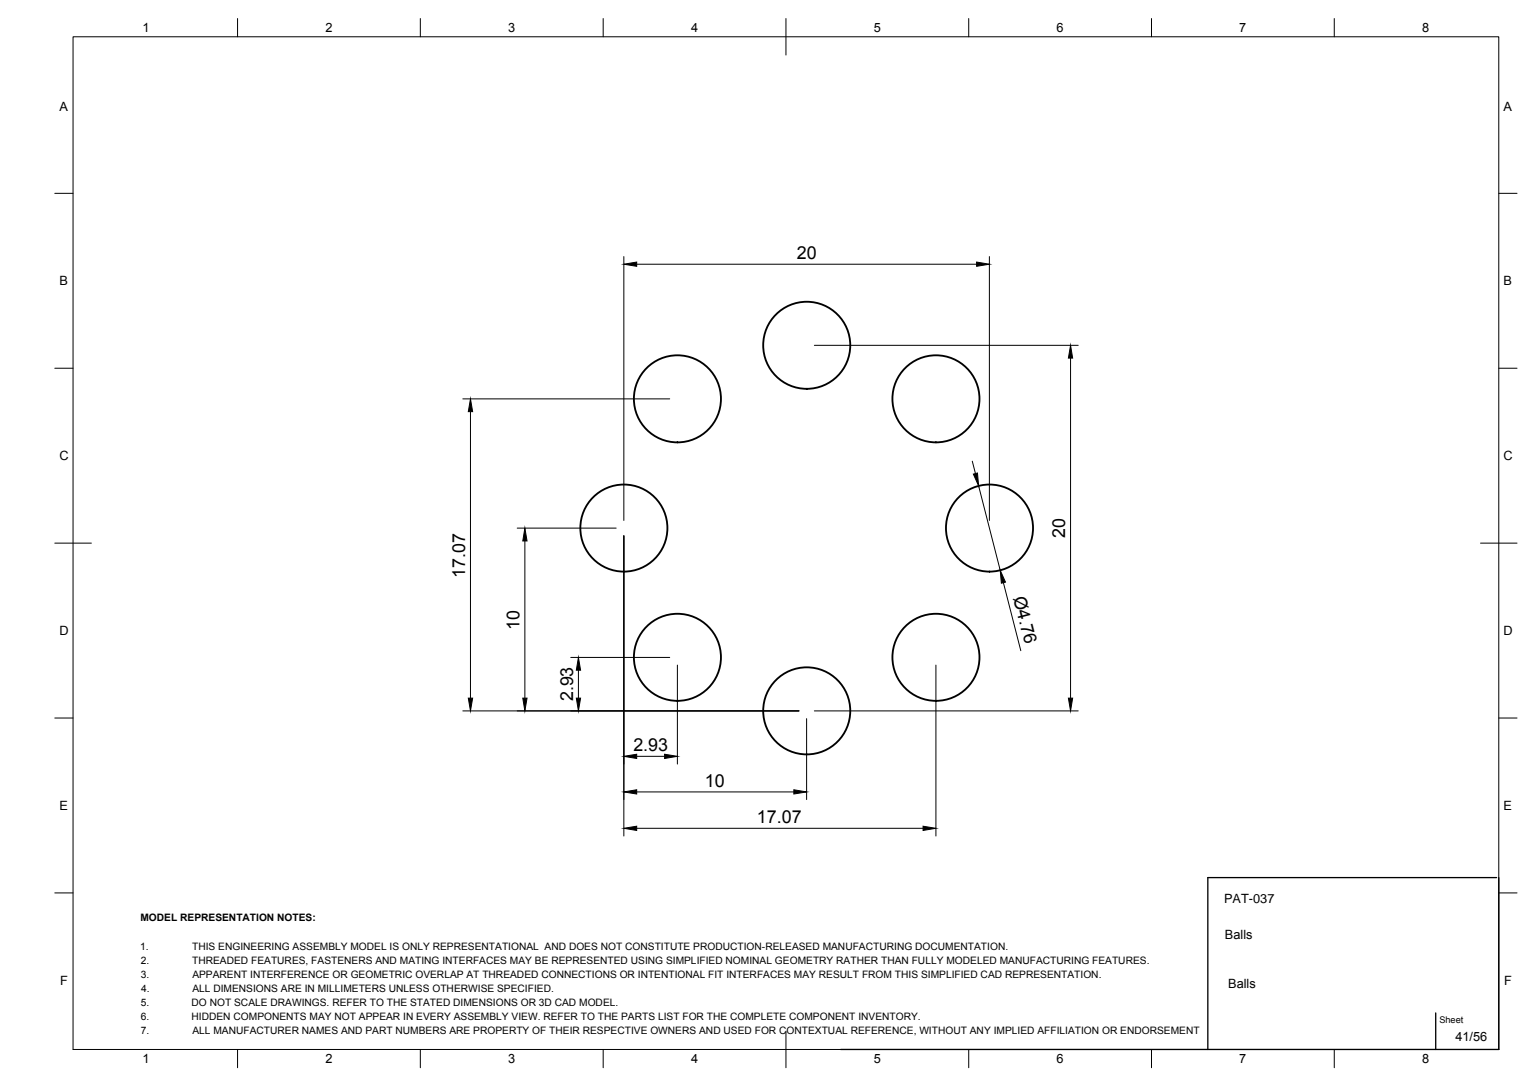
ISO-10303-21;
HEADER;
/* Generated by software containing ST-Developer
 * from STEP Tools, Inc. (www.steptools.com) 
 */

FILE_DESCRIPTION(
/* description */ ('Flywheel Crank-Slider'),
/* implementation_level */ '2;1');

FILE_NAME(
/* name */ 'Balls.step',
/* time_stamp */ '2026-10-28T03:23:13-07:00',
/* author */ (''),
/* organization */ (''),
/* preprocessor_version */ 'ST-DEVELOPER v20.2',
/* originating_system */ 'Autodesk Translation Framework v15.17.0.0',
/* authorisation */ '');

FILE_SCHEMA (('AUTOMOTIVE_DESIGN { 1 0 10303 214 3 1 1 }'));
ENDSEC;

DATA;
#10=MECHANICAL_DESIGN_GEOMETRIC_PRESENTATION_REPRESENTATION('',(#708,#709,#710,#711,#712,#713,#714,#715),#17322);
#513=SPHERICAL_SURFACE('',#10435,0.23815);
#514=SPHERICAL_SURFACE('',#10437,0.23815);
#515=SPHERICAL_SURFACE('',#10439,0.23815);
#516=SPHERICAL_SURFACE('',#10441,0.23815);
#517=SPHERICAL_SURFACE('',#10443,0.23815);
#518=SPHERICAL_SURFACE('',#10445,0.23815);
#519=SPHERICAL_SURFACE('',#10447,0.23815);
#520=SPHERICAL_SURFACE('',#10449,0.23815);
#603=SHAPE_REPRESENTATION_RELATIONSHIP('SRR','None',#17603,#655);
#655=ADVANCED_BREP_SHAPE_REPRESENTATION('',(#765,#766,#767,#768,#769,#770,
#771,#772),#17307);
#708=STYLED_ITEM('',(#17931),#765);
#709=STYLED_ITEM('',(#17931),#766);
#710=STYLED_ITEM('',(#17931),#767);
#711=STYLED_ITEM('',(#17931),#768);
#712=STYLED_ITEM('',(#17931),#769);
#713=STYLED_ITEM('',(#17931),#770);
#714=STYLED_ITEM('',(#17931),#771);
#715=STYLED_ITEM('',(#17931),#772);
#765=MANIFOLD_SOLID_BREP('Body1',#9090);
#766=MANIFOLD_SOLID_BREP('Body2',#9091);
#767=MANIFOLD_SOLID_BREP('Body3',#9092);
#768=MANIFOLD_SOLID_BREP('Body4',#9093);
#769=MANIFOLD_SOLID_BREP('Body5',#9094);
#770=MANIFOLD_SOLID_BREP('Body6',#9095);
#771=MANIFOLD_SOLID_BREP('Body7',#9096);
#772=MANIFOLD_SOLID_BREP('Body8',#9097);
#1718=FACE_OUTER_BOUND('',#2415,.T.);
#1719=FACE_OUTER_BOUND('',#2416,.T.);
#1720=FACE_OUTER_BOUND('',#2417,.T.);
#1721=FACE_OUTER_BOUND('',#2418,.T.);
#1722=FACE_OUTER_BOUND('',#2419,.T.);
#1723=FACE_OUTER_BOUND('',#2420,.T.);
#1724=FACE_OUTER_BOUND('',#2421,.T.);
#1725=FACE_OUTER_BOUND('',#2422,.T.);
#2415=EDGE_LOOP('',(#7762,#7763));
#2416=EDGE_LOOP('',(#7764,#7765));
#2417=EDGE_LOOP('',(#7766,#7767));
#2418=EDGE_LOOP('',(#7768,#7769));
#2419=EDGE_LOOP('',(#7770,#7771));
#2420=EDGE_LOOP('',(#7772,#7773));
#2421=EDGE_LOOP('',(#7774,#7775));
#2422=EDGE_LOOP('',(#7776,#7777));
#4142=CIRCLE('',#10436,0.23815);
#4143=CIRCLE('',#10438,0.23815);
#4144=CIRCLE('',#10440,0.23815);
#4145=CIRCLE('',#10442,0.23815);
#4146=CIRCLE('',#10444,0.23815);
#4147=CIRCLE('',#10446,0.23815);
#4148=CIRCLE('',#10448,0.23815);
#4149=CIRCLE('',#10450,0.23815);
#4819=VERTEX_POINT('',#16121);
#4820=VERTEX_POINT('',#16122);
#4821=VERTEX_POINT('',#16125);
#4822=VERTEX_POINT('',#16126);
#4823=VERTEX_POINT('',#16129);
#4824=VERTEX_POINT('',#16130);
#4825=VERTEX_POINT('',#16133);
#4826=VERTEX_POINT('',#16134);
#4827=VERTEX_POINT('',#16137);
#4828=VERTEX_POINT('',#16138);
#4829=VERTEX_POINT('',#16141);
#4830=VERTEX_POINT('',#16142);
#4831=VERTEX_POINT('',#16145);
#4832=VERTEX_POINT('',#16146);
#4833=VERTEX_POINT('',#16149);
#4834=VERTEX_POINT('',#16150);
#5838=EDGE_CURVE('',#4819,#4820,#4142,.T.);
#5839=EDGE_CURVE('',#4821,#4822,#4143,.T.);
#5840=EDGE_CURVE('',#4823,#4824,#4144,.T.);
#5841=EDGE_CURVE('',#4825,#4826,#4145,.T.);
#5842=EDGE_CURVE('',#4827,#4828,#4146,.T.);
#5843=EDGE_CURVE('',#4829,#4830,#4147,.T.);
#5844=EDGE_CURVE('',#4831,#4832,#4148,.T.);
#5845=EDGE_CURVE('',#4833,#4834,#4149,.T.);
#7762=ORIENTED_EDGE('',*,*,#5838,.T.);
#7763=ORIENTED_EDGE('',*,*,#5838,.F.);
#7764=ORIENTED_EDGE('',*,*,#5839,.T.);
#7765=ORIENTED_EDGE('',*,*,#5839,.F.);
#7766=ORIENTED_EDGE('',*,*,#5840,.T.);
#7767=ORIENTED_EDGE('',*,*,#5840,.F.);
#7768=ORIENTED_EDGE('',*,*,#5841,.T.);
#7769=ORIENTED_EDGE('',*,*,#5841,.F.);
#7770=ORIENTED_EDGE('',*,*,#5842,.T.);
#7771=ORIENTED_EDGE('',*,*,#5842,.F.);
#7772=ORIENTED_EDGE('',*,*,#5843,.T.);
#7773=ORIENTED_EDGE('',*,*,#5843,.F.);
#7774=ORIENTED_EDGE('',*,*,#5844,.T.);
#7775=ORIENTED_EDGE('',*,*,#5844,.F.);
#7776=ORIENTED_EDGE('',*,*,#5845,.T.);
#7777=ORIENTED_EDGE('',*,*,#5845,.F.);
#8909=ADVANCED_FACE('',(#1718),#513,.T.);
#8910=ADVANCED_FACE('',(#1719),#514,.T.);
#8911=ADVANCED_FACE('',(#1720),#515,.T.);
#8912=ADVANCED_FACE('',(#1721),#516,.T.);
#8913=ADVANCED_FACE('',(#1722),#517,.T.);
#8914=ADVANCED_FACE('',(#1723),#518,.T.);
#8915=ADVANCED_FACE('',(#1724),#519,.T.);
#8916=ADVANCED_FACE('',(#1725),#520,.T.);
#9090=CLOSED_SHELL('',(#8909));
#9091=CLOSED_SHELL('',(#8910));
#9092=CLOSED_SHELL('',(#8911));
#9093=CLOSED_SHELL('',(#8912));
#9094=CLOSED_SHELL('',(#8913));
#9095=CLOSED_SHELL('',(#8914));
#9096=CLOSED_SHELL('',(#8915));
#9097=CLOSED_SHELL('',(#8916));
#10434=AXIS2_PLACEMENT_3D('',#16119,#12808,#12809);
#10435=AXIS2_PLACEMENT_3D('',#16120,#12810,#12811);
#10436=AXIS2_PLACEMENT_3D('',#16123,#12812,#12813);
#10437=AXIS2_PLACEMENT_3D('',#16124,#12814,#12815);
#10438=AXIS2_PLACEMENT_3D('',#16127,#12816,#12817);
#10439=AXIS2_PLACEMENT_3D('',#16128,#12818,#12819);
#10440=AXIS2_PLACEMENT_3D('',#16131,#12820,#12821);
#10441=AXIS2_PLACEMENT_3D('',#16132,#12822,#12823);
#10442=AXIS2_PLACEMENT_3D('',#16135,#12824,#12825);
#10443=AXIS2_PLACEMENT_3D('',#16136,#12826,#12827);
#10444=AXIS2_PLACEMENT_3D('',#16139,#12828,#12829);
#10445=AXIS2_PLACEMENT_3D('',#16140,#12830,#12831);
#10446=AXIS2_PLACEMENT_3D('',#16143,#12832,#12833);
#10447=AXIS2_PLACEMENT_3D('',#16144,#12834,#12835);
#10448=AXIS2_PLACEMENT_3D('',#16147,#12836,#12837);
#10449=AXIS2_PLACEMENT_3D('',#16148,#12838,#12839);
#10450=AXIS2_PLACEMENT_3D('',#16151,#12840,#12841);
#12808=DIRECTION('axis',(0.,0.,1.));
#12809=DIRECTION('refdir',(1.,0.,0.));
#12810=DIRECTION('center_axis',(0.,0.,1.));
#12811=DIRECTION('ref_axis',(1.,0.,0.));
#12812=DIRECTION('center_axis',(1.22464679914735E-16,-1.,0.));
#12813=DIRECTION('ref_axis',(-1.,-1.22464679914735E-16,0.));
#12814=DIRECTION('center_axis',(0.707106781186548,0.,0.707106781186548));
#12815=DIRECTION('ref_axis',(0.707106781186548,0.,-0.707106781186548));
#12816=DIRECTION('center_axis',(8.65956056235494E-17,-1.,-8.65956056235493E-17));
#12817=DIRECTION('ref_axis',(-0.707106781186547,-1.22464679914735E-16,0.707106781186547));
#12818=DIRECTION('center_axis',(1.,0.,0.));
#12819=DIRECTION('ref_axis',(6.12323399573676E-17,0.,-1.));
#12820=DIRECTION('center_axis',(7.49879891330929E-33,-1.,-1.22464679914735E-16));
#12821=DIRECTION('ref_axis',(-6.12323399573676E-17,-1.22464679914735E-16,
1.));
#12822=DIRECTION('center_axis',(0.707106781186548,0.,-0.707106781186548));
#12823=DIRECTION('ref_axis',(-0.707106781186548,0.,-0.707106781186548));
#12824=DIRECTION('center_axis',(-8.65956056235493E-17,-1.,-8.65956056235494E-17));
#12825=DIRECTION('ref_axis',(0.707106781186547,-1.22464679914735E-16,0.707106781186547));
#12826=DIRECTION('center_axis',(0.,0.,-1.));
#12827=DIRECTION('ref_axis',(-1.,0.,-1.22464679914735E-16));
#12828=DIRECTION('center_axis',(-1.22464679914735E-16,-1.,-1.49975978266186E-32));
#12829=DIRECTION('ref_axis',(1.,-1.22464679914735E-16,1.22464679914735E-16));
#12830=DIRECTION('center_axis',(-0.707106781186547,0.,-0.707106781186548));
#12831=DIRECTION('ref_axis',(-0.707106781186548,0.,0.707106781186547));
#12832=DIRECTION('center_axis',(-8.65956056235493E-17,-1.,8.65956056235493E-17));
#12833=DIRECTION('ref_axis',(0.707106781186548,-1.22464679914735E-16,-0.707106781186547));
#12834=DIRECTION('center_axis',(-1.,0.,0.));
#12835=DIRECTION('ref_axis',(-1.83697019872103E-16,0.,1.));
#12836=DIRECTION('center_axis',(-2.24963967399279E-32,-1.,1.22464679914735E-16));
#12837=DIRECTION('ref_axis',(1.83697019872103E-16,-1.22464679914735E-16,
-1.));
#12838=DIRECTION('center_axis',(-0.707106781186548,0.,0.707106781186548));
#12839=DIRECTION('ref_axis',(0.707106781186547,0.,0.707106781186548));
#12840=DIRECTION('center_axis',(8.65956056235493E-17,-1.,8.65956056235493E-17));
#12841=DIRECTION('ref_axis',(-0.707106781186547,-1.22464679914735E-16,-0.707106781186548));
#16119=CARTESIAN_POINT('',(0.,0.,0.));
#16120=CARTESIAN_POINT('Origin',(1.,0.,0.));
#16121=CARTESIAN_POINT('',(1.,-1.78583896120461E-33,0.23815));
#16122=CARTESIAN_POINT('',(1.,-1.78583896120461E-33,-0.23815));
#16123=CARTESIAN_POINT('Origin',(1.,0.,0.));
#16124=CARTESIAN_POINT('Origin',(0.707106781186548,0.,-0.707106781186547));
#16125=CARTESIAN_POINT('',(0.875504261126124,-1.78583896120461E-33,-0.538709301246971));
#16126=CARTESIAN_POINT('',(0.538709301246971,-1.78583896120461E-33,-0.875504261126124));
#16127=CARTESIAN_POINT('Origin',(0.707106781186548,0.,-0.707106781186547));
#16128=CARTESIAN_POINT('Origin',(6.12323399573677E-17,0.,-1.));
#16129=CARTESIAN_POINT('',(0.23815,-1.78583896120461E-33,-1.));
#16130=CARTESIAN_POINT('',(-0.23815,-1.78583896120461E-33,-1.));
#16131=CARTESIAN_POINT('Origin',(6.12323399573677E-17,0.,-1.));
#16132=CARTESIAN_POINT('Origin',(-0.707106781186547,0.,-0.707106781186548));
#16133=CARTESIAN_POINT('',(-0.538709301246971,-1.78583896120461E-33,-0.875504261126124));
#16134=CARTESIAN_POINT('',(-0.875504261126124,-1.78583896120461E-33,-0.538709301246971));
#16135=CARTESIAN_POINT('Origin',(-0.707106781186547,0.,-0.707106781186548));
#16136=CARTESIAN_POINT('Origin',(-1.,0.,-1.22464679914735E-16));
#16137=CARTESIAN_POINT('',(-1.,-1.78583896120461E-33,-0.23815));
#16138=CARTESIAN_POINT('',(-1.,-1.78583896120461E-33,0.23815));
#16139=CARTESIAN_POINT('Origin',(-1.,0.,-1.22464679914735E-16));
#16140=CARTESIAN_POINT('Origin',(-0.707106781186548,0.,0.707106781186547));
#16141=CARTESIAN_POINT('',(-0.875504261126124,-7.94881478324376E-33,0.538709301246971));
#16142=CARTESIAN_POINT('',(-0.538709301246971,4.37713686083455E-33,0.875504261126124));
#16143=CARTESIAN_POINT('Origin',(-0.707106781186548,0.,0.707106781186547));
#16144=CARTESIAN_POINT('Origin',(-1.83697019872103E-16,0.,1.));
#16145=CARTESIAN_POINT('',(-0.23815,-1.78583896120461E-33,1.));
#16146=CARTESIAN_POINT('',(0.23815,-1.78583896120461E-33,1.));
#16147=CARTESIAN_POINT('Origin',(-1.83697019872103E-16,0.,1.));
#16148=CARTESIAN_POINT('Origin',(0.707106781186547,0.,0.707106781186548));
#16149=CARTESIAN_POINT('',(0.538709301246971,-4.86732687222419E-33,0.875504261126124));
#16150=CARTESIAN_POINT('',(0.875504261126124,1.29564894981497E-33,0.538709301246971));
#16151=CARTESIAN_POINT('Origin',(0.707106781186547,0.,0.707106781186548));
#17246=UNCERTAINTY_MEASURE_WITH_UNIT(LENGTH_MEASURE(0.001),#17323,
'DISTANCE_ACCURACY_VALUE',
'Maximum model space distance between geometric entities at asserted c
onnectivities');
#17261=UNCERTAINTY_MEASURE_WITH_UNIT(LENGTH_MEASURE(0.001),#17323,
'DISTANCE_ACCURACY_VALUE',
'Maximum model space distance between geometric entities at asserted c
onnectivities');
#17307=(
GEOMETRIC_REPRESENTATION_CONTEXT(3)
GLOBAL_UNCERTAINTY_ASSIGNED_CONTEXT((#17246))
GLOBAL_UNIT_ASSIGNED_CONTEXT((#17323,#17325,#17326))
REPRESENTATION_CONTEXT('','3D')
);
#17322=(
GEOMETRIC_REPRESENTATION_CONTEXT(3)
GLOBAL_UNCERTAINTY_ASSIGNED_CONTEXT((#17261))
GLOBAL_UNIT_ASSIGNED_CONTEXT((#17323,#17325,#17326))
REPRESENTATION_CONTEXT('','3D')
);
#17323=(
LENGTH_UNIT()
NAMED_UNIT(*)
SI_UNIT(.CENTI.,.METRE.)
);
#17325=(
NAMED_UNIT(*)
PLANE_ANGLE_UNIT()
SI_UNIT($,.RADIAN.)
);
#17326=(
NAMED_UNIT(*)
SI_UNIT($,.STERADIAN.)
SOLID_ANGLE_UNIT()
);
#17372=SHAPE_DEFINITION_REPRESENTATION(#17434,#17603);
#17434=PRODUCT_DEFINITION_SHAPE('',$,#17664);
#17603=SHAPE_REPRESENTATION('',(#10434),#17307);
#17618=PRODUCT_DEFINITION_CONTEXT('part definition',#17800,'design');
#17664=PRODUCT_DEFINITION('Balls','Balls',#17724,#17618);
#17724=PRODUCT_DEFINITION_FORMATION('',$,#17847);
#17800=APPLICATION_CONTEXT(
'Core Data for Automotive Mechanical Design Process');
#17801=PRODUCT_CONTEXT('part definition',#17800,'mechanical');
#17847=PRODUCT('Balls','Balls','Balls',(#17801));
#17925=COLOUR_RGB('Grey',0.48,0.52,0.57);
#17926=FILL_AREA_STYLE_COLOUR('',#17925);
#17927=FILL_AREA_STYLE('',(#17926));
#17928=SURFACE_STYLE_FILL_AREA(#17927);
#17929=SURFACE_SIDE_STYLE('',(#17928));
#17930=SURFACE_STYLE_USAGE(.BOTH.,#17929);
#17931=PRESENTATION_STYLE_ASSIGNMENT((#17930));
ENDSEC;
END-ISO-10303-21;
